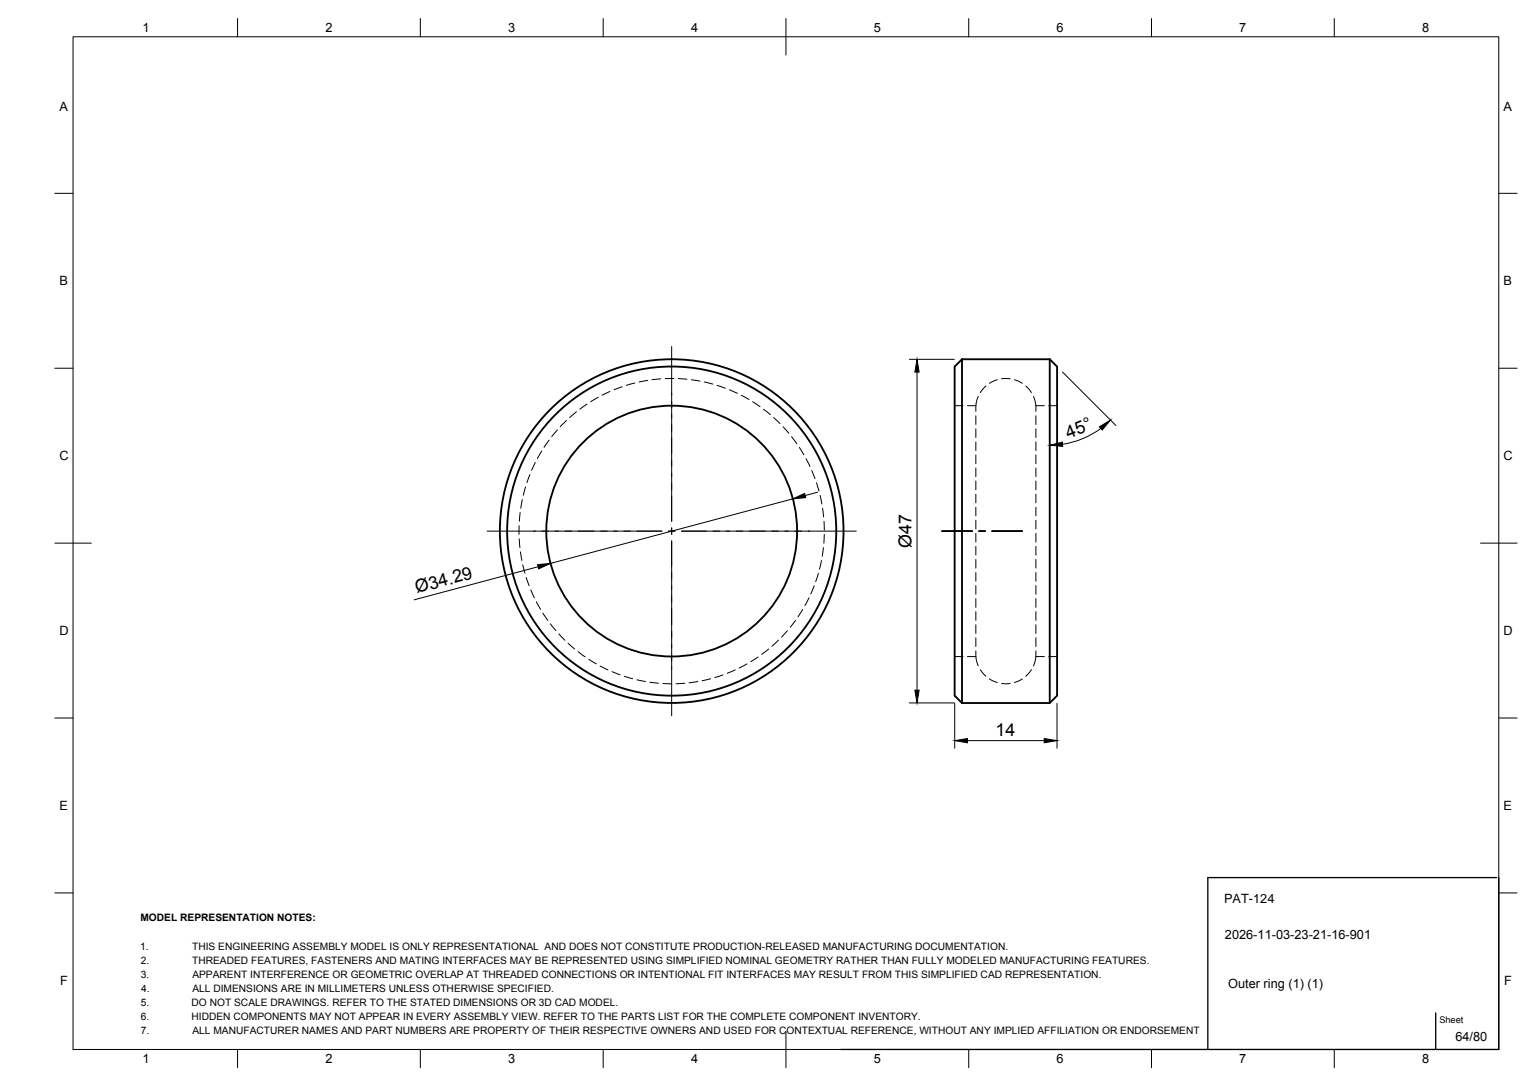
ISO-10303-21;
HEADER;
/* Generated by software containing ST-Developer
 * from STEP Tools, Inc. (www.steptools.com) 
 */

FILE_DESCRIPTION(
/* description */ ('XY cross-slide table'),
/* implementation_level */ '2;1');

FILE_NAME(
/* name */ 'Outer ring (1) (1).step',
/* time_stamp */ '2026-10-28T03:22:46-07:00',
/* author */ (''),
/* organization */ (''),
/* preprocessor_version */ 'ST-DEVELOPER v20.2',
/* originating_system */ 'Autodesk Translation Framework v15.17.0.0',
/* authorisation */ '');

FILE_SCHEMA (('AUTOMOTIVE_DESIGN { 1 0 10303 214 3 1 1 }'));
ENDSEC;

DATA;
#10=MECHANICAL_DESIGN_GEOMETRIC_PRESENTATION_REPRESENTATION('',(#1749),#62984);
#1473=CONICAL_SURFACE('',#25691,2.3,0.785398163397449);
#1474=CONICAL_SURFACE('',#25695,2.3,0.785398163397449);
#1503=TOROIDAL_SURFACE('',#25680,1.675,0.412776);
#1561=SHAPE_REPRESENTATION_RELATIONSHIP('SRR','None',#63418,#1644);
#1644=ADVANCED_BREP_SHAPE_REPRESENTATION('',(#1858),#62955);
#1749=STYLED_ITEM('',(#63912),#1858);
#1858=MANIFOLD_SOLID_BREP('Body1',#23047);
#2212=FACE_BOUND('',#5373,.T.);
#2213=FACE_BOUND('',#5378,.T.);
#2680=PLANE('',#25688);
#2681=PLANE('',#25697);
#3731=FACE_OUTER_BOUND('',#5370,.T.);
#3732=FACE_OUTER_BOUND('',#5371,.T.);
#3733=FACE_OUTER_BOUND('',#5372,.T.);
#3734=FACE_OUTER_BOUND('',#5374,.T.);
#3735=FACE_OUTER_BOUND('',#5375,.T.);
#3736=FACE_OUTER_BOUND('',#5376,.T.);
#3737=FACE_OUTER_BOUND('',#5377,.T.);
#3738=FACE_OUTER_BOUND('',#5379,.T.);
#5370=EDGE_LOOP('',(#18858,#18859,#18860,#18861,#18862,#18863));
#5371=EDGE_LOOP('',(#18864,#18865,#18866,#18867,#18868));
#5372=EDGE_LOOP('',(#18869));
#5373=EDGE_LOOP('',(#18870));
#5374=EDGE_LOOP('',(#18871,#18872,#18873,#18874));
#5375=EDGE_LOOP('',(#18875,#18876,#18877,#18878));
#5376=EDGE_LOOP('',(#18879,#18880,#18881,#18882));
#5377=EDGE_LOOP('',(#18883));
#5378=EDGE_LOOP('',(#18884));
#5379=EDGE_LOOP('',(#18885,#18886,#18887,#18888,#18889));
#6858=LINE('',#49108,#8345);
#6859=LINE('',#49117,#8346);
#6860=LINE('',#49121,#8347);
#6861=LINE('',#49125,#8348);
#6862=LINE('',#49128,#8349);
#8345=VECTOR('',#30789,1.71469);
#8346=VECTOR('',#30800,2.3);
#8347=VECTOR('',#30805,2.35);
#8348=VECTOR('',#30810,2.3);
#8349=VECTOR('',#30815,1.71469);
#9547=CIRCLE('',#25681,1.71469);
#9548=CIRCLE('',#25682,1.71469);
#9549=CIRCLE('',#25683,0.412776);
#9550=CIRCLE('',#25684,1.71469);
#9551=CIRCLE('',#25685,1.71469);
#9552=CIRCLE('',#25687,1.71469);
#9553=CIRCLE('',#25689,2.25);
#9554=CIRCLE('',#25690,1.71469);
#9555=CIRCLE('',#25692,2.35);
#9556=CIRCLE('',#25694,2.35);
#9557=CIRCLE('',#25696,2.25);
#11105=VERTEX_POINT('',#49096);
#11106=VERTEX_POINT('',#49097);
#11107=VERTEX_POINT('',#49100);
#11108=VERTEX_POINT('',#49102);
#11109=VERTEX_POINT('',#49106);
#11110=VERTEX_POINT('',#49110);
#11111=VERTEX_POINT('',#49112);
#11112=VERTEX_POINT('',#49115);
#11113=VERTEX_POINT('',#49119);
#11114=VERTEX_POINT('',#49123);
#13813=EDGE_CURVE('',#11105,#11106,#9547,.T.);
#13814=EDGE_CURVE('',#11106,#11105,#9548,.T.);
#13815=EDGE_CURVE('',#11106,#11107,#9549,.T.);
#13816=EDGE_CURVE('',#11108,#11107,#9550,.T.);
#13817=EDGE_CURVE('',#11107,#11108,#9551,.T.);
#13818=EDGE_CURVE('',#11109,#11109,#9552,.T.);
#13819=EDGE_CURVE('',#11109,#11108,#6858,.T.);
#13820=EDGE_CURVE('',#11110,#11110,#9553,.T.);
#13821=EDGE_CURVE('',#11111,#11111,#9554,.T.);
#13822=EDGE_CURVE('',#11112,#11112,#9555,.T.);
#13823=EDGE_CURVE('',#11112,#11110,#6859,.T.);
#13824=EDGE_CURVE('',#11113,#11113,#9556,.T.);
#13825=EDGE_CURVE('',#11113,#11112,#6860,.T.);
#13826=EDGE_CURVE('',#11114,#11114,#9557,.T.);
#13827=EDGE_CURVE('',#11114,#11113,#6861,.T.);
#13828=EDGE_CURVE('',#11105,#11111,#6862,.T.);
#18858=ORIENTED_EDGE('',*,*,#13813,.F.);
#18859=ORIENTED_EDGE('',*,*,#13814,.F.);
#18860=ORIENTED_EDGE('',*,*,#13815,.T.);
#18861=ORIENTED_EDGE('',*,*,#13816,.F.);
#18862=ORIENTED_EDGE('',*,*,#13817,.F.);
#18863=ORIENTED_EDGE('',*,*,#13815,.F.);
#18864=ORIENTED_EDGE('',*,*,#13818,.T.);
#18865=ORIENTED_EDGE('',*,*,#13819,.T.);
#18866=ORIENTED_EDGE('',*,*,#13816,.T.);
#18867=ORIENTED_EDGE('',*,*,#13817,.T.);
#18868=ORIENTED_EDGE('',*,*,#13819,.F.);
#18869=ORIENTED_EDGE('',*,*,#13820,.F.);
#18870=ORIENTED_EDGE('',*,*,#13821,.T.);
#18871=ORIENTED_EDGE('',*,*,#13822,.F.);
#18872=ORIENTED_EDGE('',*,*,#13823,.T.);
#18873=ORIENTED_EDGE('',*,*,#13820,.T.);
#18874=ORIENTED_EDGE('',*,*,#13823,.F.);
#18875=ORIENTED_EDGE('',*,*,#13824,.F.);
#18876=ORIENTED_EDGE('',*,*,#13825,.T.);
#18877=ORIENTED_EDGE('',*,*,#13822,.T.);
#18878=ORIENTED_EDGE('',*,*,#13825,.F.);
#18879=ORIENTED_EDGE('',*,*,#13826,.F.);
#18880=ORIENTED_EDGE('',*,*,#13827,.T.);
#18881=ORIENTED_EDGE('',*,*,#13824,.T.);
#18882=ORIENTED_EDGE('',*,*,#13827,.F.);
#18883=ORIENTED_EDGE('',*,*,#13826,.T.);
#18884=ORIENTED_EDGE('',*,*,#13818,.F.);
#18885=ORIENTED_EDGE('',*,*,#13813,.T.);
#18886=ORIENTED_EDGE('',*,*,#13814,.T.);
#18887=ORIENTED_EDGE('',*,*,#13828,.T.);
#18888=ORIENTED_EDGE('',*,*,#13821,.F.);
#18889=ORIENTED_EDGE('',*,*,#13828,.F.);
#21431=CYLINDRICAL_SURFACE('',#25686,1.71469);
#21432=CYLINDRICAL_SURFACE('',#25693,2.35);
#21433=CYLINDRICAL_SURFACE('',#25698,1.71469);
#22512=ADVANCED_FACE('',(#3731),#1503,.F.);
#22513=ADVANCED_FACE('',(#3732),#21431,.F.);
#22514=ADVANCED_FACE('',(#3733,#2212),#2680,.T.);
#22515=ADVANCED_FACE('',(#3734),#1473,.T.);
#22516=ADVANCED_FACE('',(#3735),#21432,.T.);
#22517=ADVANCED_FACE('',(#3736),#1474,.T.);
#22518=ADVANCED_FACE('',(#3737,#2213),#2681,.T.);
#22519=ADVANCED_FACE('',(#3738),#21433,.F.);
#23047=CLOSED_SHELL('',(#22512,#22513,#22514,#22515,#22516,#22517,#22518,
#22519));
#25679=AXIS2_PLACEMENT_3D('',#49094,#30771,#30772);
#25680=AXIS2_PLACEMENT_3D('',#49095,#30773,#30774);
#25681=AXIS2_PLACEMENT_3D('',#49098,#30775,#30776);
#25682=AXIS2_PLACEMENT_3D('',#49099,#30777,#30778);
#25683=AXIS2_PLACEMENT_3D('',#49101,#30779,#30780);
#25684=AXIS2_PLACEMENT_3D('',#49103,#30781,#30782);
#25685=AXIS2_PLACEMENT_3D('',#49104,#30783,#30784);
#25686=AXIS2_PLACEMENT_3D('',#49105,#30785,#30786);
#25687=AXIS2_PLACEMENT_3D('',#49107,#30787,#30788);
#25688=AXIS2_PLACEMENT_3D('',#49109,#30790,#30791);
#25689=AXIS2_PLACEMENT_3D('',#49111,#30792,#30793);
#25690=AXIS2_PLACEMENT_3D('',#49113,#30794,#30795);
#25691=AXIS2_PLACEMENT_3D('',#49114,#30796,#30797);
#25692=AXIS2_PLACEMENT_3D('',#49116,#30798,#30799);
#25693=AXIS2_PLACEMENT_3D('',#49118,#30801,#30802);
#25694=AXIS2_PLACEMENT_3D('',#49120,#30803,#30804);
#25695=AXIS2_PLACEMENT_3D('',#49122,#30806,#30807);
#25696=AXIS2_PLACEMENT_3D('',#49124,#30808,#30809);
#25697=AXIS2_PLACEMENT_3D('',#49126,#30811,#30812);
#25698=AXIS2_PLACEMENT_3D('',#49127,#30813,#30814);
#30771=DIRECTION('axis',(0.,0.,1.));
#30772=DIRECTION('refdir',(1.,0.,0.));
#30773=DIRECTION('center_axis',(0.,-1.,0.));
#30774=DIRECTION('ref_axis',(0.,0.,-1.));
#30775=DIRECTION('center_axis',(0.,-1.,0.));
#30776=DIRECTION('ref_axis',(1.,0.,0.));
#30777=DIRECTION('center_axis',(0.,-1.,0.));
#30778=DIRECTION('ref_axis',(1.,0.,0.));
#30779=DIRECTION('center_axis',(1.,0.,1.22464679914735E-16));
#30780=DIRECTION('ref_axis',(-1.22464679914735E-16,0.,1.));
#30781=DIRECTION('center_axis',(0.,1.,0.));
#30782=DIRECTION('ref_axis',(1.,0.,0.));
#30783=DIRECTION('center_axis',(0.,1.,0.));
#30784=DIRECTION('ref_axis',(1.,0.,0.));
#30785=DIRECTION('center_axis',(0.,-1.,0.));
#30786=DIRECTION('ref_axis',(1.,0.,0.));
#30787=DIRECTION('center_axis',(0.,-1.,0.));
#30788=DIRECTION('ref_axis',(1.,0.,0.));
#30789=DIRECTION('',(0.,1.,0.));
#30790=DIRECTION('center_axis',(0.,1.,0.));
#30791=DIRECTION('ref_axis',(0.,0.,1.));
#30792=DIRECTION('center_axis',(0.,-1.,0.));
#30793=DIRECTION('ref_axis',(1.,0.,0.));
#30794=DIRECTION('center_axis',(0.,-1.,0.));
#30795=DIRECTION('ref_axis',(1.,0.,0.));
#30796=DIRECTION('center_axis',(0.,-1.,0.));
#30797=DIRECTION('ref_axis',(1.,0.,0.));
#30798=DIRECTION('center_axis',(0.,-1.,0.));
#30799=DIRECTION('ref_axis',(1.,0.,0.));
#30800=DIRECTION('',(0.707106781186548,0.707106781186547,8.65956056235494E-17));
#30801=DIRECTION('center_axis',(0.,-1.,0.));
#30802=DIRECTION('ref_axis',(1.,0.,0.));
#30803=DIRECTION('center_axis',(0.,-1.,0.));
#30804=DIRECTION('ref_axis',(1.,0.,0.));
#30805=DIRECTION('',(0.,1.,0.));
#30806=DIRECTION('center_axis',(0.,1.,0.));
#30807=DIRECTION('ref_axis',(1.,0.,0.));
#30808=DIRECTION('center_axis',(0.,-1.,0.));
#30809=DIRECTION('ref_axis',(1.,0.,0.));
#30810=DIRECTION('',(-0.707106781186548,0.707106781186547,-8.65956056235494E-17));
#30811=DIRECTION('center_axis',(0.,-1.,0.));
#30812=DIRECTION('ref_axis',(0.,0.,-1.));
#30813=DIRECTION('center_axis',(0.,-1.,0.));
#30814=DIRECTION('ref_axis',(1.,0.,0.));
#30815=DIRECTION('',(0.,1.,0.));
#49094=CARTESIAN_POINT('',(0.,0.,0.));
#49095=CARTESIAN_POINT('Origin',(0.,0.,0.));
#49096=CARTESIAN_POINT('',(-1.71469,0.410863395882378,-2.09988962002998E-16));
#49097=CARTESIAN_POINT('',(-2.09988962002998E-16,0.410863395882378,1.71469));
#49098=CARTESIAN_POINT('Origin',(0.,0.410863395882378,0.));
#49099=CARTESIAN_POINT('Origin',(0.,0.410863395882378,0.));
#49100=CARTESIAN_POINT('',(-2.09988962002998E-16,-0.410863395882378,1.71469));
#49101=CARTESIAN_POINT('Origin',(-2.05128338857182E-16,0.,1.675));
#49102=CARTESIAN_POINT('',(-1.71469,-0.410863395882378,2.09988962002998E-16));
#49103=CARTESIAN_POINT('Origin',(0.,-0.410863395882378,0.));
#49104=CARTESIAN_POINT('Origin',(0.,-0.410863395882378,0.));
#49105=CARTESIAN_POINT('Origin',(0.,0.,0.));
#49106=CARTESIAN_POINT('',(-1.71469,-0.7,-2.09988962002998E-16));
#49107=CARTESIAN_POINT('Origin',(0.,-0.7,0.));
#49108=CARTESIAN_POINT('',(-1.71469,0.,-2.09988962002998E-16));
#49109=CARTESIAN_POINT('Origin',(2.25,0.7,0.));
#49110=CARTESIAN_POINT('',(-2.25,0.7,-2.75545529808154E-16));
#49111=CARTESIAN_POINT('Origin',(0.,0.7,0.));
#49112=CARTESIAN_POINT('',(-1.71469,0.7,-2.09988962002998E-16));
#49113=CARTESIAN_POINT('Origin',(0.,0.7,0.));
#49114=CARTESIAN_POINT('Origin',(0.,0.65,0.));
#49115=CARTESIAN_POINT('',(-2.35,0.6,-2.87791997799628E-16));
#49116=CARTESIAN_POINT('Origin',(0.,0.6,0.));
#49117=CARTESIAN_POINT('',(-2.3,0.65,-2.81668763803891E-16));
#49118=CARTESIAN_POINT('Origin',(0.,0.,0.));
#49119=CARTESIAN_POINT('',(-2.35,-0.6,-2.87791997799628E-16));
#49120=CARTESIAN_POINT('Origin',(0.,-0.6,0.));
#49121=CARTESIAN_POINT('',(-2.35,0.,-2.87791997799628E-16));
#49122=CARTESIAN_POINT('Origin',(0.,-0.65,0.));
#49123=CARTESIAN_POINT('',(-2.25,-0.7,-2.75545529808154E-16));
#49124=CARTESIAN_POINT('Origin',(0.,-0.7,0.));
#49125=CARTESIAN_POINT('',(-2.3,-0.65,-2.81668763803891E-16));
#49126=CARTESIAN_POINT('Origin',(1.71469,-0.7,0.));
#49127=CARTESIAN_POINT('Origin',(0.,0.,0.));
#49128=CARTESIAN_POINT('',(-1.71469,0.,-2.09988962002998E-16));
#62856=UNCERTAINTY_MEASURE_WITH_UNIT(LENGTH_MEASURE(0.001),#62985,
'DISTANCE_ACCURACY_VALUE',
'Maximum model space distance between geometric entities at asserted c
onnectivities');
#62885=UNCERTAINTY_MEASURE_WITH_UNIT(LENGTH_MEASURE(0.001),#62985,
'DISTANCE_ACCURACY_VALUE',
'Maximum model space distance between geometric entities at asserted c
onnectivities');
#62955=(
GEOMETRIC_REPRESENTATION_CONTEXT(3)
GLOBAL_UNCERTAINTY_ASSIGNED_CONTEXT((#62856))
GLOBAL_UNIT_ASSIGNED_CONTEXT((#62985,#62987,#62988))
REPRESENTATION_CONTEXT('','3D')
);
#62984=(
GEOMETRIC_REPRESENTATION_CONTEXT(3)
GLOBAL_UNCERTAINTY_ASSIGNED_CONTEXT((#62885))
GLOBAL_UNIT_ASSIGNED_CONTEXT((#62985,#62987,#62988))
REPRESENTATION_CONTEXT('','3D')
);
#62985=(
LENGTH_UNIT()
NAMED_UNIT(*)
SI_UNIT(.CENTI.,.METRE.)
);
#62987=(
NAMED_UNIT(*)
PLANE_ANGLE_UNIT()
SI_UNIT($,.RADIAN.)
);
#62988=(
NAMED_UNIT(*)
SI_UNIT($,.STERADIAN.)
SOLID_ANGLE_UNIT()
);
#63058=SHAPE_DEFINITION_REPRESENTATION(#63241,#63418);
#63241=PRODUCT_DEFINITION_SHAPE('',$,#63517);
#63418=SHAPE_REPRESENTATION('',(#25679),#62955);
#63447=PRODUCT_DEFINITION_CONTEXT('part definition',#63743,'design');
#63517=PRODUCT_DEFINITION('Outer ring (1) (1)','Outer ring (1) (1)',#63615,
#63447);
#63615=PRODUCT_DEFINITION_FORMATION('',$,#63814);
#63743=APPLICATION_CONTEXT(
'Core Data for Automotive Mechanical Design Process');
#63744=PRODUCT_CONTEXT('part definition',#63743,'mechanical');
#63814=PRODUCT('Outer ring (1) (1)','Outer ring (1) (1)','Outer ring (1) (1)',(#63744));
#63906=COLOUR_RGB('Grey',0.48,0.52,0.57);
#63907=FILL_AREA_STYLE_COLOUR('',#63906);
#63908=FILL_AREA_STYLE('',(#63907));
#63909=SURFACE_STYLE_FILL_AREA(#63908);
#63910=SURFACE_SIDE_STYLE('',(#63909));
#63911=SURFACE_STYLE_USAGE(.BOTH.,#63910);
#63912=PRESENTATION_STYLE_ASSIGNMENT((#63911));
ENDSEC;
END-ISO-10303-21;
